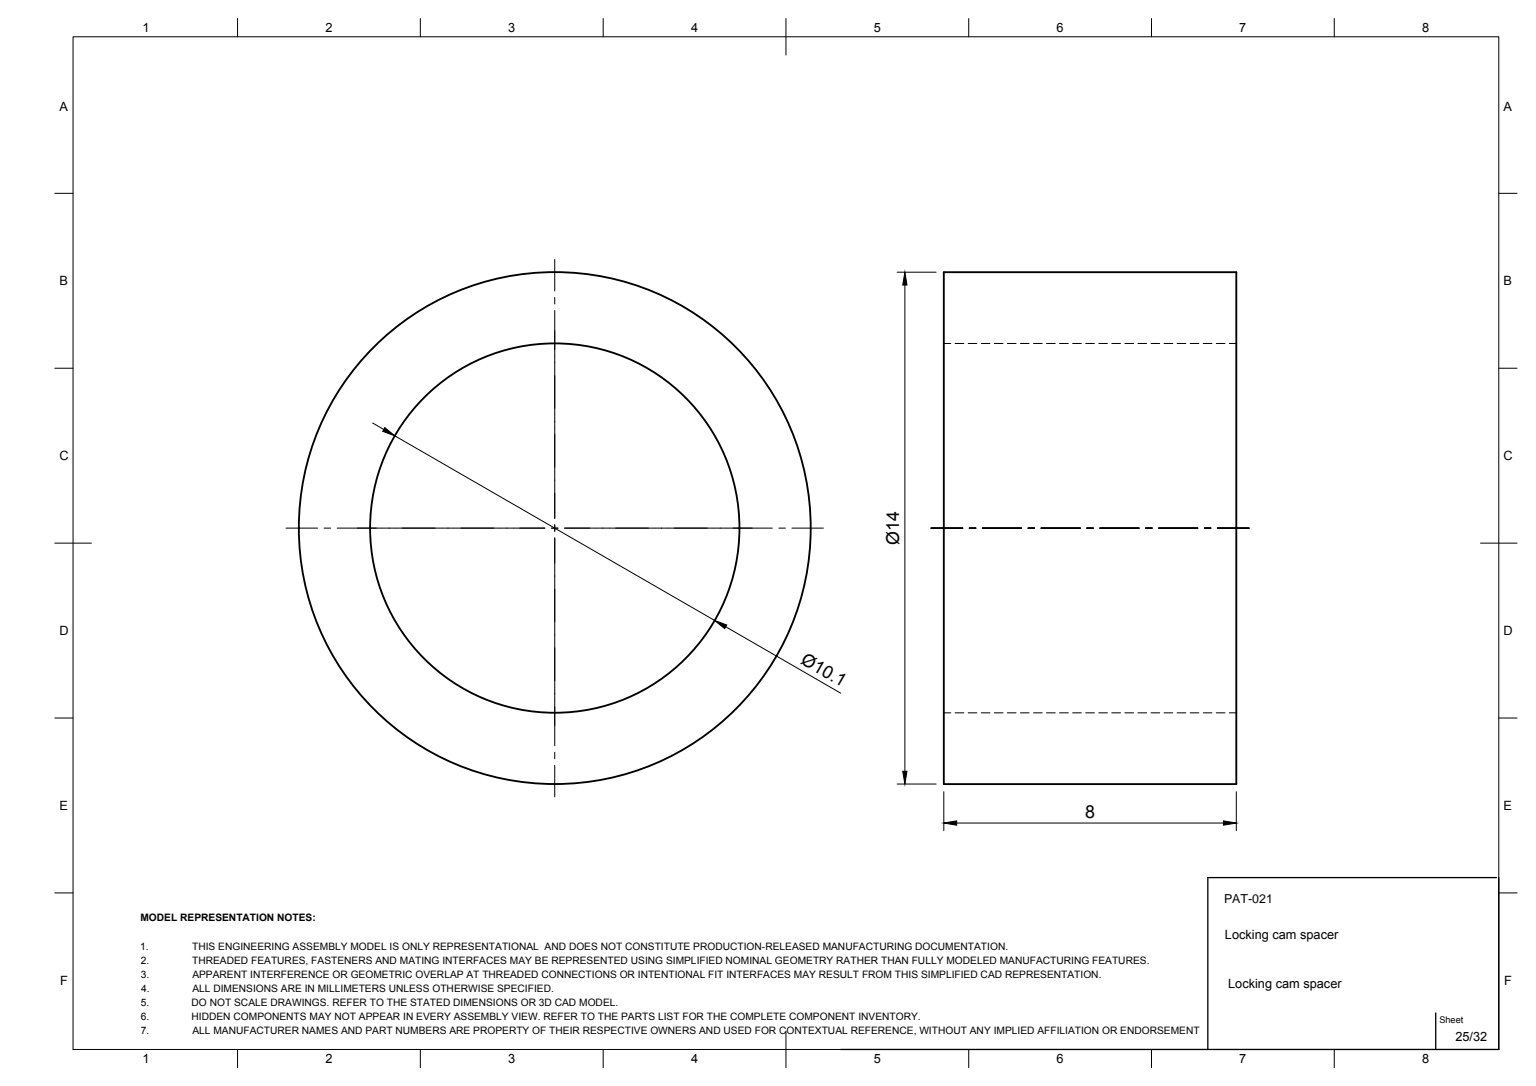
ISO-10303-21;
HEADER;
/* Generated by software containing ST-Developer
 * from STEP Tools, Inc. (www.steptools.com) 
 */

FILE_DESCRIPTION(
/* description */ ('Chain-less indexing wheel (Geneva) drive'),
/* implementation_level */ '2;1');

FILE_NAME(
/* name */ 'Locking cam spacer.step',
/* time_stamp */ '2026-10-28T03:25:22-07:00',
/* author */ (''),
/* organization */ (''),
/* preprocessor_version */ 'ST-DEVELOPER v20.2',
/* originating_system */ 'Autodesk Translation Framework v15.17.0.0',
/* authorisation */ '');

FILE_SCHEMA (('AUTOMOTIVE_DESIGN { 1 0 10303 214 3 1 1 }'));
ENDSEC;

DATA;
#10=MECHANICAL_DESIGN_GEOMETRIC_PRESENTATION_REPRESENTATION('',(#328),#10957);
#270=SHAPE_REPRESENTATION_RELATIONSHIP('SRR','None',#11085,#295);
#295=ADVANCED_BREP_SHAPE_REPRESENTATION('',(#360),#10948);
#328=STYLED_ITEM('',(#11301),#360);
#360=MANIFOLD_SOLID_BREP('Body1',#5725);
#449=FACE_BOUND('',#1293,.T.);
#450=FACE_BOUND('',#1295,.T.);
#583=PLANE('',#6505);
#584=PLANE('',#6506);
#875=FACE_OUTER_BOUND('',#1290,.T.);
#876=FACE_OUTER_BOUND('',#1291,.T.);
#877=FACE_OUTER_BOUND('',#1292,.T.);
#878=FACE_OUTER_BOUND('',#1294,.T.);
#1290=EDGE_LOOP('',(#4707,#4708,#4709,#4710));
#1291=EDGE_LOOP('',(#4711,#4712,#4713,#4714));
#1292=EDGE_LOOP('',(#4715));
#1293=EDGE_LOOP('',(#4716));
#1294=EDGE_LOOP('',(#4717));
#1295=EDGE_LOOP('',(#4718));
#1634=LINE('',#10178,#2008);
#1635=LINE('',#10184,#2009);
#2008=VECTOR('',#7942,0.505);
#2009=VECTOR('',#7949,0.7);
#2410=CIRCLE('',#6500,0.505);
#2411=CIRCLE('',#6501,0.505);
#2412=CIRCLE('',#6503,0.7);
#2413=CIRCLE('',#6504,0.7);
#2822=VERTEX_POINT('',#10175);
#2823=VERTEX_POINT('',#10177);
#2824=VERTEX_POINT('',#10181);
#2825=VERTEX_POINT('',#10183);
#3479=EDGE_CURVE('',#2822,#2822,#2410,.T.);
#3480=EDGE_CURVE('',#2822,#2823,#1634,.T.);
#3481=EDGE_CURVE('',#2823,#2823,#2411,.T.);
#3482=EDGE_CURVE('',#2824,#2824,#2412,.T.);
#3483=EDGE_CURVE('',#2824,#2825,#1635,.T.);
#3484=EDGE_CURVE('',#2825,#2825,#2413,.T.);
#4707=ORIENTED_EDGE('',*,*,#3479,.F.);
#4708=ORIENTED_EDGE('',*,*,#3480,.T.);
#4709=ORIENTED_EDGE('',*,*,#3481,.T.);
#4710=ORIENTED_EDGE('',*,*,#3480,.F.);
#4711=ORIENTED_EDGE('',*,*,#3482,.F.);
#4712=ORIENTED_EDGE('',*,*,#3483,.T.);
#4713=ORIENTED_EDGE('',*,*,#3484,.T.);
#4714=ORIENTED_EDGE('',*,*,#3483,.F.);
#4715=ORIENTED_EDGE('',*,*,#3482,.T.);
#4716=ORIENTED_EDGE('',*,*,#3479,.T.);
#4717=ORIENTED_EDGE('',*,*,#3484,.F.);
#4718=ORIENTED_EDGE('',*,*,#3481,.F.);
#5329=CYLINDRICAL_SURFACE('',#6499,0.505);
#5330=CYLINDRICAL_SURFACE('',#6502,0.7);
#5589=ADVANCED_FACE('',(#875),#5329,.F.);
#5590=ADVANCED_FACE('',(#876),#5330,.T.);
#5591=ADVANCED_FACE('',(#877,#449),#583,.T.);
#5592=ADVANCED_FACE('',(#878,#450),#584,.F.);
#5725=CLOSED_SHELL('',(#5589,#5590,#5591,#5592));
#6498=AXIS2_PLACEMENT_3D('',#10173,#7936,#7937);
#6499=AXIS2_PLACEMENT_3D('',#10174,#7938,#7939);
#6500=AXIS2_PLACEMENT_3D('',#10176,#7940,#7941);
#6501=AXIS2_PLACEMENT_3D('',#10179,#7943,#7944);
#6502=AXIS2_PLACEMENT_3D('',#10180,#7945,#7946);
#6503=AXIS2_PLACEMENT_3D('',#10182,#7947,#7948);
#6504=AXIS2_PLACEMENT_3D('',#10185,#7950,#7951);
#6505=AXIS2_PLACEMENT_3D('',#10186,#7952,#7953);
#6506=AXIS2_PLACEMENT_3D('',#10187,#7954,#7955);
#7936=DIRECTION('axis',(0.,0.,1.));
#7937=DIRECTION('refdir',(1.,0.,0.));
#7938=DIRECTION('center_axis',(0.,0.,1.));
#7939=DIRECTION('ref_axis',(1.,0.,0.));
#7940=DIRECTION('center_axis',(0.,0.,-1.));
#7941=DIRECTION('ref_axis',(1.,0.,0.));
#7942=DIRECTION('',(0.,0.,-1.));
#7943=DIRECTION('center_axis',(0.,0.,-1.));
#7944=DIRECTION('ref_axis',(1.,0.,0.));
#7945=DIRECTION('center_axis',(0.,0.,1.));
#7946=DIRECTION('ref_axis',(1.,0.,0.));
#7947=DIRECTION('center_axis',(0.,0.,1.));
#7948=DIRECTION('ref_axis',(1.,0.,0.));
#7949=DIRECTION('',(0.,0.,-1.));
#7950=DIRECTION('center_axis',(0.,0.,1.));
#7951=DIRECTION('ref_axis',(1.,0.,0.));
#7952=DIRECTION('center_axis',(0.,0.,1.));
#7953=DIRECTION('ref_axis',(1.,0.,0.));
#7954=DIRECTION('center_axis',(0.,0.,1.));
#7955=DIRECTION('ref_axis',(1.,0.,0.));
#10173=CARTESIAN_POINT('',(0.,0.,0.));
#10174=CARTESIAN_POINT('Origin',(0.,0.,5.2));
#10175=CARTESIAN_POINT('',(-0.505,-6.18446633569413E-17,6.));
#10176=CARTESIAN_POINT('Origin',(0.,0.,6.));
#10177=CARTESIAN_POINT('',(-0.505,-6.18446633569413E-17,5.2));
#10178=CARTESIAN_POINT('',(-0.505,-6.18446633569413E-17,5.2));
#10179=CARTESIAN_POINT('Origin',(0.,0.,5.2));
#10180=CARTESIAN_POINT('Origin',(0.,0.,5.2));
#10181=CARTESIAN_POINT('',(-0.7,-8.57252759403147E-17,6.));
#10182=CARTESIAN_POINT('Origin',(0.,0.,6.));
#10183=CARTESIAN_POINT('',(-0.7,-8.57252759403147E-17,5.2));
#10184=CARTESIAN_POINT('',(-0.7,-8.57252759403147E-17,5.2));
#10185=CARTESIAN_POINT('Origin',(0.,0.,5.2));
#10186=CARTESIAN_POINT('Origin',(0.,0.,6.));
#10187=CARTESIAN_POINT('Origin',(0.,0.,5.2));
#10917=UNCERTAINTY_MEASURE_WITH_UNIT(LENGTH_MEASURE(0.001),#10958,
'DISTANCE_ACCURACY_VALUE',
'Maximum model space distance between geometric entities at asserted c
onnectivities');
#10926=UNCERTAINTY_MEASURE_WITH_UNIT(LENGTH_MEASURE(0.001),#10958,
'DISTANCE_ACCURACY_VALUE',
'Maximum model space distance between geometric entities at asserted c
onnectivities');
#10948=(
GEOMETRIC_REPRESENTATION_CONTEXT(3)
GLOBAL_UNCERTAINTY_ASSIGNED_CONTEXT((#10917))
GLOBAL_UNIT_ASSIGNED_CONTEXT((#10958,#10960,#10961))
REPRESENTATION_CONTEXT('','3D')
);
#10957=(
GEOMETRIC_REPRESENTATION_CONTEXT(3)
GLOBAL_UNCERTAINTY_ASSIGNED_CONTEXT((#10926))
GLOBAL_UNIT_ASSIGNED_CONTEXT((#10958,#10960,#10961))
REPRESENTATION_CONTEXT('','3D')
);
#10958=(
LENGTH_UNIT()
NAMED_UNIT(*)
SI_UNIT(.CENTI.,.METRE.)
);
#10960=(
NAMED_UNIT(*)
PLANE_ANGLE_UNIT()
SI_UNIT($,.RADIAN.)
);
#10961=(
NAMED_UNIT(*)
SI_UNIT($,.STERADIAN.)
SOLID_ANGLE_UNIT()
);
#10983=SHAPE_DEFINITION_REPRESENTATION(#11018,#11085);
#11018=PRODUCT_DEFINITION_SHAPE('',$,#11116);
#11085=SHAPE_REPRESENTATION('',(#6498),#10948);
#11094=PRODUCT_DEFINITION_CONTEXT('part definition',#11186,'design');
#11116=PRODUCT_DEFINITION('Locking cam spacer','Locking cam spacer',#11146,
#11094);
#11146=PRODUCT_DEFINITION_FORMATION('',$,#11209);
#11186=APPLICATION_CONTEXT(
'Core Data for Automotive Mechanical Design Process');
#11187=PRODUCT_CONTEXT('part definition',#11186,'mechanical');
#11209=PRODUCT('Locking cam spacer','Locking cam spacer',
'Locking cam spacer',(#11187));
#11295=COLOUR_RGB('Off White',0.89,0.88,0.83);
#11296=FILL_AREA_STYLE_COLOUR('',#11295);
#11297=FILL_AREA_STYLE('',(#11296));
#11298=SURFACE_STYLE_FILL_AREA(#11297);
#11299=SURFACE_SIDE_STYLE('',(#11298));
#11300=SURFACE_STYLE_USAGE(.BOTH.,#11299);
#11301=PRESENTATION_STYLE_ASSIGNMENT((#11300));
ENDSEC;
END-ISO-10303-21;
